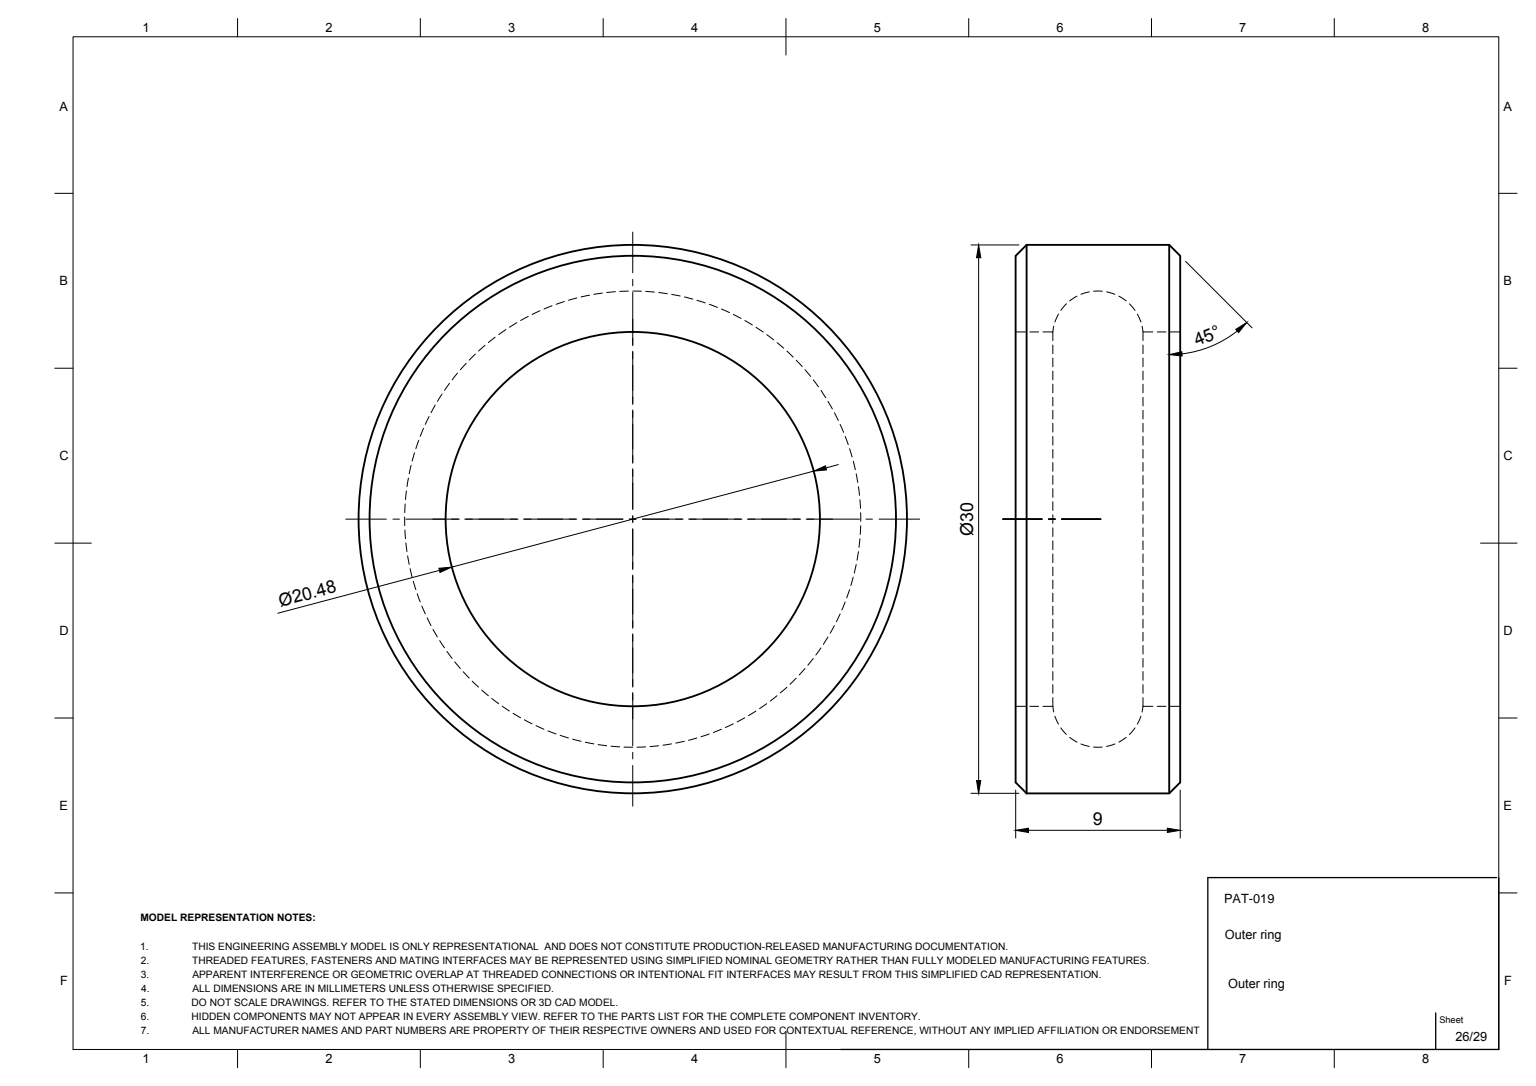
ISO-10303-21;
HEADER;
/* Generated by software containing ST-Developer
 * from STEP Tools, Inc. (www.steptools.com) 
 */

FILE_DESCRIPTION(
/* description */ ('Caster wheel assembly'),
/* implementation_level */ '2;1');

FILE_NAME(
/* name */ 'Outer ring.step',
/* time_stamp */ '2026-10-28T03:23:56-07:00',
/* author */ (''),
/* organization */ (''),
/* preprocessor_version */ 'ST-DEVELOPER v20.2',
/* originating_system */ 'Autodesk Translation Framework v15.17.0.0',
/* authorisation */ '');

FILE_SCHEMA (('AUTOMOTIVE_DESIGN { 1 0 10303 214 3 1 1 }'));
ENDSEC;

DATA;
#10=MECHANICAL_DESIGN_GEOMETRIC_PRESENTATION_REPRESENTATION('',(#240),#5385);
#46=TOROIDAL_SURFACE('',#3184,1.,0.247676);
#176=CONICAL_SURFACE('',#3195,1.47,0.785398163397449);
#177=CONICAL_SURFACE('',#3199,1.47,0.785398163397449);
#196=SHAPE_REPRESENTATION_RELATIONSHIP('SRR','None',#5494,#218);
#218=ADVANCED_BREP_SHAPE_REPRESENTATION('',(#269),#5381);
#240=STYLED_ITEM('',(#5672),#269);
#269=MANIFOLD_SOLID_BREP('Body1',#2668);
#326=FACE_BOUND('',#762,.T.);
#327=FACE_BOUND('',#767,.T.);
#406=PLANE('',#3192);
#407=PLANE('',#3201);
#546=FACE_OUTER_BOUND('',#759,.T.);
#547=FACE_OUTER_BOUND('',#760,.T.);
#548=FACE_OUTER_BOUND('',#761,.T.);
#549=FACE_OUTER_BOUND('',#763,.T.);
#550=FACE_OUTER_BOUND('',#764,.T.);
#551=FACE_OUTER_BOUND('',#765,.T.);
#552=FACE_OUTER_BOUND('',#766,.T.);
#553=FACE_OUTER_BOUND('',#768,.T.);
#759=EDGE_LOOP('',(#2248,#2249,#2250,#2251,#2252,#2253));
#760=EDGE_LOOP('',(#2254,#2255,#2256,#2257,#2258));
#761=EDGE_LOOP('',(#2259));
#762=EDGE_LOOP('',(#2260));
#763=EDGE_LOOP('',(#2261,#2262,#2263,#2264));
#764=EDGE_LOOP('',(#2265,#2266,#2267,#2268));
#765=EDGE_LOOP('',(#2269,#2270,#2271,#2272));
#766=EDGE_LOOP('',(#2273));
#767=EDGE_LOOP('',(#2274));
#768=EDGE_LOOP('',(#2275,#2276,#2277,#2278,#2279));
#932=LINE('',#4786,#1066);
#933=LINE('',#4795,#1067);
#934=LINE('',#4799,#1068);
#935=LINE('',#4803,#1069);
#936=LINE('',#4806,#1070);
#1066=VECTOR('',#3965,1.023815);
#1067=VECTOR('',#3976,1.47);
#1068=VECTOR('',#3981,1.5);
#1069=VECTOR('',#3986,1.47);
#1070=VECTOR('',#3991,1.023815);
#1175=CIRCLE('',#3185,1.023815);
#1176=CIRCLE('',#3186,1.023815);
#1177=CIRCLE('',#3187,0.247676);
#1178=CIRCLE('',#3188,1.023815);
#1179=CIRCLE('',#3189,1.023815);
#1180=CIRCLE('',#3191,1.023815);
#1181=CIRCLE('',#3193,1.44);
#1182=CIRCLE('',#3194,1.023815);
#1183=CIRCLE('',#3196,1.5);
#1184=CIRCLE('',#3198,1.5);
#1185=CIRCLE('',#3200,1.44);
#1389=VERTEX_POINT('',#4774);
#1390=VERTEX_POINT('',#4775);
#1391=VERTEX_POINT('',#4778);
#1392=VERTEX_POINT('',#4780);
#1393=VERTEX_POINT('',#4784);
#1394=VERTEX_POINT('',#4788);
#1395=VERTEX_POINT('',#4790);
#1396=VERTEX_POINT('',#4793);
#1397=VERTEX_POINT('',#4797);
#1398=VERTEX_POINT('',#4801);
#1692=EDGE_CURVE('',#1389,#1390,#1175,.T.);
#1693=EDGE_CURVE('',#1390,#1389,#1176,.T.);
#1694=EDGE_CURVE('',#1390,#1391,#1177,.T.);
#1695=EDGE_CURVE('',#1392,#1391,#1178,.T.);
#1696=EDGE_CURVE('',#1391,#1392,#1179,.T.);
#1697=EDGE_CURVE('',#1393,#1393,#1180,.T.);
#1698=EDGE_CURVE('',#1393,#1392,#932,.T.);
#1699=EDGE_CURVE('',#1394,#1394,#1181,.T.);
#1700=EDGE_CURVE('',#1395,#1395,#1182,.T.);
#1701=EDGE_CURVE('',#1396,#1396,#1183,.T.);
#1702=EDGE_CURVE('',#1396,#1394,#933,.T.);
#1703=EDGE_CURVE('',#1397,#1397,#1184,.T.);
#1704=EDGE_CURVE('',#1397,#1396,#934,.T.);
#1705=EDGE_CURVE('',#1398,#1398,#1185,.T.);
#1706=EDGE_CURVE('',#1398,#1397,#935,.T.);
#1707=EDGE_CURVE('',#1389,#1395,#936,.T.);
#2248=ORIENTED_EDGE('',*,*,#1692,.F.);
#2249=ORIENTED_EDGE('',*,*,#1693,.F.);
#2250=ORIENTED_EDGE('',*,*,#1694,.T.);
#2251=ORIENTED_EDGE('',*,*,#1695,.F.);
#2252=ORIENTED_EDGE('',*,*,#1696,.F.);
#2253=ORIENTED_EDGE('',*,*,#1694,.F.);
#2254=ORIENTED_EDGE('',*,*,#1697,.T.);
#2255=ORIENTED_EDGE('',*,*,#1698,.T.);
#2256=ORIENTED_EDGE('',*,*,#1695,.T.);
#2257=ORIENTED_EDGE('',*,*,#1696,.T.);
#2258=ORIENTED_EDGE('',*,*,#1698,.F.);
#2259=ORIENTED_EDGE('',*,*,#1699,.F.);
#2260=ORIENTED_EDGE('',*,*,#1700,.T.);
#2261=ORIENTED_EDGE('',*,*,#1701,.F.);
#2262=ORIENTED_EDGE('',*,*,#1702,.T.);
#2263=ORIENTED_EDGE('',*,*,#1699,.T.);
#2264=ORIENTED_EDGE('',*,*,#1702,.F.);
#2265=ORIENTED_EDGE('',*,*,#1703,.F.);
#2266=ORIENTED_EDGE('',*,*,#1704,.T.);
#2267=ORIENTED_EDGE('',*,*,#1701,.T.);
#2268=ORIENTED_EDGE('',*,*,#1704,.F.);
#2269=ORIENTED_EDGE('',*,*,#1705,.F.);
#2270=ORIENTED_EDGE('',*,*,#1706,.T.);
#2271=ORIENTED_EDGE('',*,*,#1703,.T.);
#2272=ORIENTED_EDGE('',*,*,#1706,.F.);
#2273=ORIENTED_EDGE('',*,*,#1705,.T.);
#2274=ORIENTED_EDGE('',*,*,#1697,.F.);
#2275=ORIENTED_EDGE('',*,*,#1692,.T.);
#2276=ORIENTED_EDGE('',*,*,#1693,.T.);
#2277=ORIENTED_EDGE('',*,*,#1707,.T.);
#2278=ORIENTED_EDGE('',*,*,#1700,.F.);
#2279=ORIENTED_EDGE('',*,*,#1707,.F.);
#2472=CYLINDRICAL_SURFACE('',#3190,1.023815);
#2473=CYLINDRICAL_SURFACE('',#3197,1.5);
#2474=CYLINDRICAL_SURFACE('',#3202,1.023815);
#2606=ADVANCED_FACE('',(#546),#46,.F.);
#2607=ADVANCED_FACE('',(#547),#2472,.F.);
#2608=ADVANCED_FACE('',(#548,#326),#406,.T.);
#2609=ADVANCED_FACE('',(#549),#176,.T.);
#2610=ADVANCED_FACE('',(#550),#2473,.T.);
#2611=ADVANCED_FACE('',(#551),#177,.T.);
#2612=ADVANCED_FACE('',(#552,#327),#407,.T.);
#2613=ADVANCED_FACE('',(#553),#2474,.F.);
#2668=CLOSED_SHELL('',(#2606,#2607,#2608,#2609,#2610,#2611,#2612,#2613));
#3183=AXIS2_PLACEMENT_3D('',#4772,#3947,#3948);
#3184=AXIS2_PLACEMENT_3D('',#4773,#3949,#3950);
#3185=AXIS2_PLACEMENT_3D('',#4776,#3951,#3952);
#3186=AXIS2_PLACEMENT_3D('',#4777,#3953,#3954);
#3187=AXIS2_PLACEMENT_3D('',#4779,#3955,#3956);
#3188=AXIS2_PLACEMENT_3D('',#4781,#3957,#3958);
#3189=AXIS2_PLACEMENT_3D('',#4782,#3959,#3960);
#3190=AXIS2_PLACEMENT_3D('',#4783,#3961,#3962);
#3191=AXIS2_PLACEMENT_3D('',#4785,#3963,#3964);
#3192=AXIS2_PLACEMENT_3D('',#4787,#3966,#3967);
#3193=AXIS2_PLACEMENT_3D('',#4789,#3968,#3969);
#3194=AXIS2_PLACEMENT_3D('',#4791,#3970,#3971);
#3195=AXIS2_PLACEMENT_3D('',#4792,#3972,#3973);
#3196=AXIS2_PLACEMENT_3D('',#4794,#3974,#3975);
#3197=AXIS2_PLACEMENT_3D('',#4796,#3977,#3978);
#3198=AXIS2_PLACEMENT_3D('',#4798,#3979,#3980);
#3199=AXIS2_PLACEMENT_3D('',#4800,#3982,#3983);
#3200=AXIS2_PLACEMENT_3D('',#4802,#3984,#3985);
#3201=AXIS2_PLACEMENT_3D('',#4804,#3987,#3988);
#3202=AXIS2_PLACEMENT_3D('',#4805,#3989,#3990);
#3947=DIRECTION('axis',(0.,0.,1.));
#3948=DIRECTION('refdir',(1.,0.,0.));
#3949=DIRECTION('center_axis',(0.,-1.,0.));
#3950=DIRECTION('ref_axis',(0.,0.,-1.));
#3951=DIRECTION('center_axis',(0.,-1.,0.));
#3952=DIRECTION('ref_axis',(1.,0.,0.));
#3953=DIRECTION('center_axis',(0.,-1.,0.));
#3954=DIRECTION('ref_axis',(1.,0.,0.));
#3955=DIRECTION('center_axis',(1.,0.,1.22464679914735E-16));
#3956=DIRECTION('ref_axis',(-1.22464679914735E-16,0.,1.));
#3957=DIRECTION('center_axis',(0.,1.,0.));
#3958=DIRECTION('ref_axis',(1.,0.,0.));
#3959=DIRECTION('center_axis',(0.,1.,0.));
#3960=DIRECTION('ref_axis',(1.,0.,0.));
#3961=DIRECTION('center_axis',(0.,-1.,0.));
#3962=DIRECTION('ref_axis',(1.,0.,0.));
#3963=DIRECTION('center_axis',(0.,-1.,0.));
#3964=DIRECTION('ref_axis',(1.,0.,0.));
#3965=DIRECTION('',(0.,1.,0.));
#3966=DIRECTION('center_axis',(0.,1.,0.));
#3967=DIRECTION('ref_axis',(0.,0.,1.));
#3968=DIRECTION('center_axis',(0.,-1.,0.));
#3969=DIRECTION('ref_axis',(1.,0.,0.));
#3970=DIRECTION('center_axis',(0.,-1.,0.));
#3971=DIRECTION('ref_axis',(1.,0.,0.));
#3972=DIRECTION('center_axis',(0.,-1.,0.));
#3973=DIRECTION('ref_axis',(1.,0.,0.));
#3974=DIRECTION('center_axis',(0.,-1.,0.));
#3975=DIRECTION('ref_axis',(1.,0.,0.));
#3976=DIRECTION('',(0.707106781186548,0.707106781186547,8.65956056235494E-17));
#3977=DIRECTION('center_axis',(0.,-1.,0.));
#3978=DIRECTION('ref_axis',(1.,0.,0.));
#3979=DIRECTION('center_axis',(0.,-1.,0.));
#3980=DIRECTION('ref_axis',(1.,0.,0.));
#3981=DIRECTION('',(0.,1.,0.));
#3982=DIRECTION('center_axis',(0.,1.,0.));
#3983=DIRECTION('ref_axis',(1.,0.,0.));
#3984=DIRECTION('center_axis',(0.,-1.,0.));
#3985=DIRECTION('ref_axis',(1.,0.,0.));
#3986=DIRECTION('',(-0.707106781186548,0.707106781186547,-8.65956056235494E-17));
#3987=DIRECTION('center_axis',(0.,-1.,0.));
#3988=DIRECTION('ref_axis',(0.,0.,-1.));
#3989=DIRECTION('center_axis',(0.,-1.,0.));
#3990=DIRECTION('ref_axis',(1.,0.,0.));
#3991=DIRECTION('',(0.,1.,0.));
#4772=CARTESIAN_POINT('',(0.,0.,0.));
#4773=CARTESIAN_POINT('Origin',(0.,0.,0.));
#4774=CARTESIAN_POINT('',(-1.023815,0.246528389340863,-1.25381176266905E-16));
#4775=CARTESIAN_POINT('',(-1.25381176266905E-16,0.246528389340863,1.023815));
#4776=CARTESIAN_POINT('Origin',(0.,0.246528389340863,0.));
#4777=CARTESIAN_POINT('Origin',(0.,0.246528389340863,0.));
#4778=CARTESIAN_POINT('',(-1.25381176266905E-16,-0.246528389340863,1.023815));
#4779=CARTESIAN_POINT('Origin',(-1.22464679914735E-16,0.,1.));
#4780=CARTESIAN_POINT('',(-1.023815,-0.246528389340863,1.25381176266905E-16));
#4781=CARTESIAN_POINT('Origin',(0.,-0.246528389340863,0.));
#4782=CARTESIAN_POINT('Origin',(0.,-0.246528389340863,0.));
#4783=CARTESIAN_POINT('Origin',(0.,0.,0.));
#4784=CARTESIAN_POINT('',(-1.023815,-0.45,-1.25381176266905E-16));
#4785=CARTESIAN_POINT('Origin',(0.,-0.45,0.));
#4786=CARTESIAN_POINT('',(-1.023815,0.,-1.25381176266905E-16));
#4787=CARTESIAN_POINT('Origin',(1.44,0.45,0.));
#4788=CARTESIAN_POINT('',(-1.44,0.45,-1.76349139077219E-16));
#4789=CARTESIAN_POINT('Origin',(0.,0.45,0.));
#4790=CARTESIAN_POINT('',(-1.023815,0.45,-1.25381176266905E-16));
#4791=CARTESIAN_POINT('Origin',(0.,0.45,0.));
#4792=CARTESIAN_POINT('Origin',(0.,0.42,0.));
#4793=CARTESIAN_POINT('',(-1.5,0.39,-1.83697019872103E-16));
#4794=CARTESIAN_POINT('Origin',(0.,0.39,0.));
#4795=CARTESIAN_POINT('',(-1.47,0.42,-1.80023079474661E-16));
#4796=CARTESIAN_POINT('Origin',(0.,0.,0.));
#4797=CARTESIAN_POINT('',(-1.5,-0.39,-1.83697019872103E-16));
#4798=CARTESIAN_POINT('Origin',(0.,-0.39,0.));
#4799=CARTESIAN_POINT('',(-1.5,0.,-1.83697019872103E-16));
#4800=CARTESIAN_POINT('Origin',(0.,-0.42,0.));
#4801=CARTESIAN_POINT('',(-1.44,-0.45,-1.76349139077219E-16));
#4802=CARTESIAN_POINT('Origin',(0.,-0.45,0.));
#4803=CARTESIAN_POINT('',(-1.47,-0.42,-1.80023079474661E-16));
#4804=CARTESIAN_POINT('Origin',(1.023815,-0.45,0.));
#4805=CARTESIAN_POINT('Origin',(0.,0.,0.));
#4806=CARTESIAN_POINT('',(-1.023815,0.,-1.25381176266905E-16));
#5353=UNCERTAINTY_MEASURE_WITH_UNIT(LENGTH_MEASURE(0.001),#5386,
'DISTANCE_ACCURACY_VALUE',
'Maximum model space distance between geometric entities at asserted c
onnectivities');
#5357=UNCERTAINTY_MEASURE_WITH_UNIT(LENGTH_MEASURE(0.001),#5386,
'DISTANCE_ACCURACY_VALUE',
'Maximum model space distance between geometric entities at asserted c
onnectivities');
#5381=(
GEOMETRIC_REPRESENTATION_CONTEXT(3)
GLOBAL_UNCERTAINTY_ASSIGNED_CONTEXT((#5353))
GLOBAL_UNIT_ASSIGNED_CONTEXT((#5386,#5388,#5389))
REPRESENTATION_CONTEXT('','3D')
);
#5385=(
GEOMETRIC_REPRESENTATION_CONTEXT(3)
GLOBAL_UNCERTAINTY_ASSIGNED_CONTEXT((#5357))
GLOBAL_UNIT_ASSIGNED_CONTEXT((#5386,#5388,#5389))
REPRESENTATION_CONTEXT('','3D')
);
#5386=(
LENGTH_UNIT()
NAMED_UNIT(*)
SI_UNIT(.CENTI.,.METRE.)
);
#5388=(
NAMED_UNIT(*)
PLANE_ANGLE_UNIT()
SI_UNIT($,.RADIAN.)
);
#5389=(
NAMED_UNIT(*)
SI_UNIT($,.STERADIAN.)
SOLID_ANGLE_UNIT()
);
#5413=SHAPE_DEFINITION_REPRESENTATION(#5454,#5494);
#5454=PRODUCT_DEFINITION_SHAPE('',$,#5522);
#5494=SHAPE_REPRESENTATION('',(#3183),#5381);
#5498=PRODUCT_DEFINITION_CONTEXT('part definition',#5581,'design');
#5522=PRODUCT_DEFINITION('Outer ring','Outer ring',#5549,#5498);
#5549=PRODUCT_DEFINITION_FORMATION('',$,#5606);
#5581=APPLICATION_CONTEXT(
'Core Data for Automotive Mechanical Design Process');
#5582=PRODUCT_CONTEXT('part definition',#5581,'mechanical');
#5606=PRODUCT('Outer ring','Outer ring','Outer ring',(#5582));
#5666=COLOUR_RGB('Grey',0.48,0.52,0.57);
#5667=FILL_AREA_STYLE_COLOUR('',#5666);
#5668=FILL_AREA_STYLE('',(#5667));
#5669=SURFACE_STYLE_FILL_AREA(#5668);
#5670=SURFACE_SIDE_STYLE('',(#5669));
#5671=SURFACE_STYLE_USAGE(.BOTH.,#5670);
#5672=PRESENTATION_STYLE_ASSIGNMENT((#5671));
ENDSEC;
END-ISO-10303-21;
